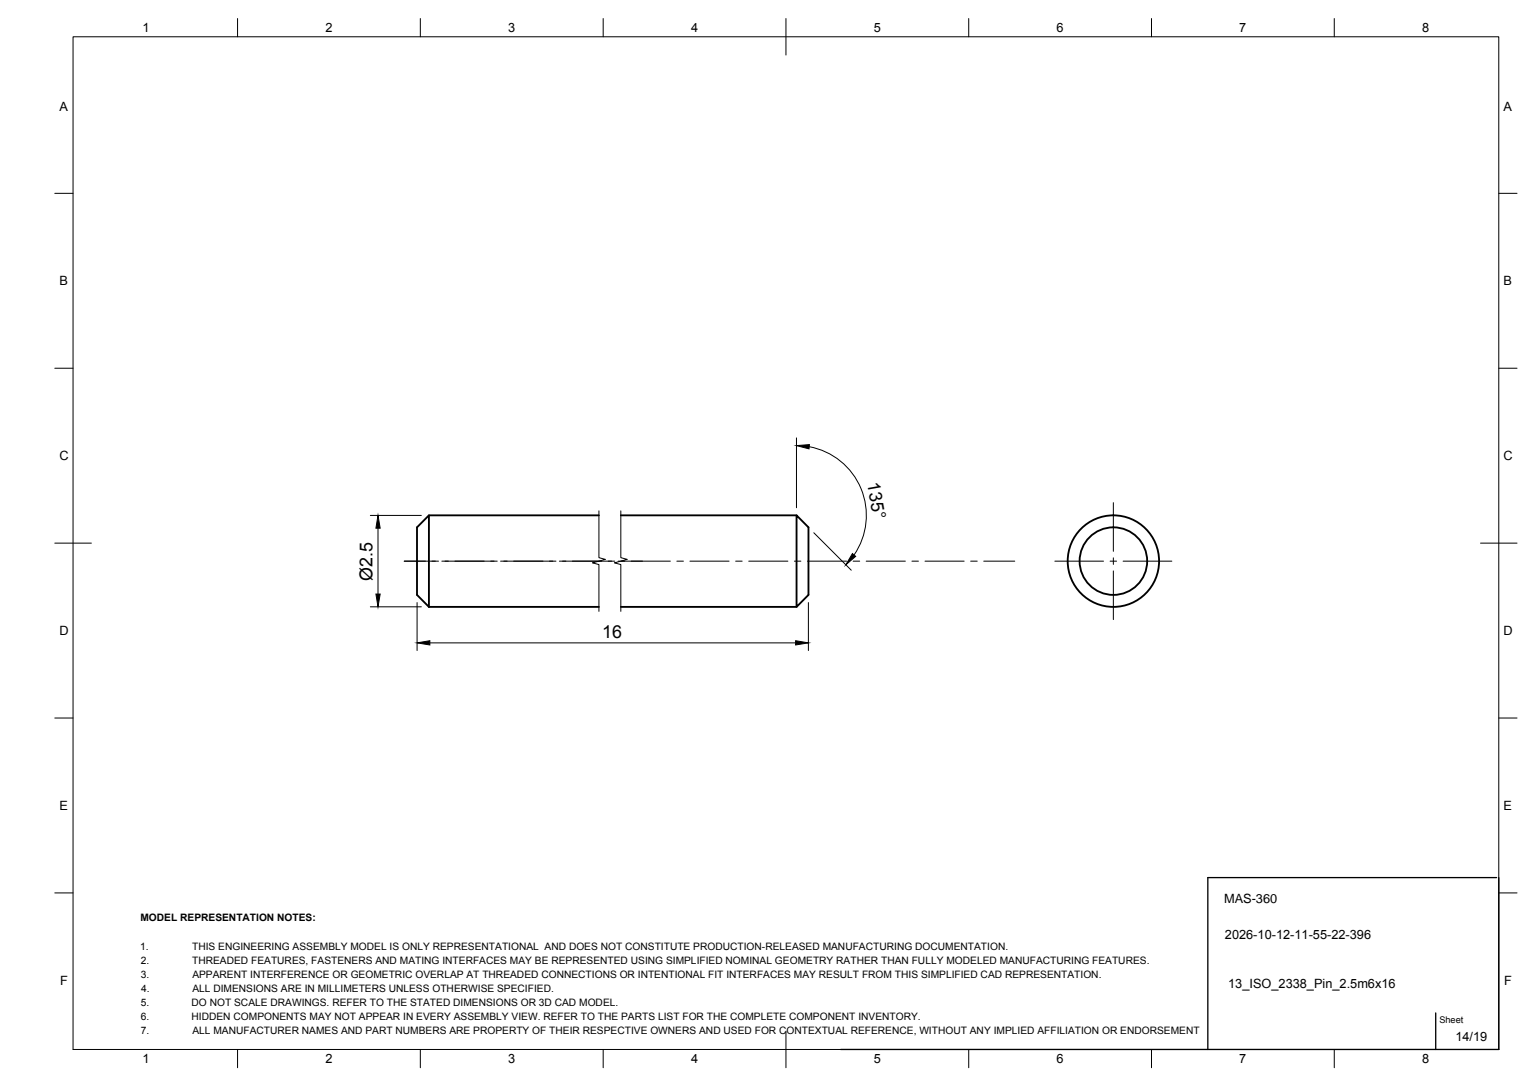
ISO-10303-21;
HEADER;
/* Generated by software containing ST-Developer
 * from STEP Tools, Inc. (www.steptools.com) 
 */

FILE_DESCRIPTION(
/* description */ (''),
/* implementation_level */ '2;1');

FILE_NAME(
/* name */ '13_ISO_2338_Pin_2.5m6x16.step',
/* time_stamp */ '2026-11-04T18:53:29-08:00',
/* author */ (''),
/* organization */ (''),
/* preprocessor_version */ 'ST-DEVELOPER v20.2',
/* originating_system */ 'Autodesk Translation Framework v15.17.0.0',
/* authorisation */ '');

FILE_SCHEMA (('AUTOMOTIVE_DESIGN { 1 0 10303 214 3 1 1 }'));
ENDSEC;

DATA;
#10=MECHANICAL_DESIGN_GEOMETRIC_PRESENTATION_REPRESENTATION('',(#1340),#100031);
#241=CONICAL_SURFACE('',#22428,1.0868,0.785398163397447);
#242=CONICAL_SURFACE('',#22433,1.0868,0.785398163397447);
#1152=CIRCLE('',#22429,1.25);
#1153=CIRCLE('',#22430,0.9236);
#1154=CIRCLE('',#22432,1.25);
#1155=CIRCLE('',#22434,0.9236);
#1304=SHAPE_REPRESENTATION_RELATIONSHIP('SRR','None',#100114,#1322);
#1322=ADVANCED_BREP_SHAPE_REPRESENTATION('',(#1358),#100026);
#1340=STYLED_ITEM('',(#100203),#1358);
#1358=MANIFOLD_SOLID_BREP('Body1',#20130);
#1679=PLANE('',#22435);
#1680=PLANE('',#22436);
#3248=LINE('',#99849,#4535);
#3249=LINE('',#99854,#4536);
#3250=LINE('',#99857,#4537);
#4535=VECTOR('',#27985,1.0868);
#4536=VECTOR('',#27992,1.25);
#4537=VECTOR('',#27995,1.0868);
#5016=CYLINDRICAL_SURFACE('',#22431,1.25);
#6147=FACE_OUTER_BOUND('',#7414,.T.);
#6148=FACE_OUTER_BOUND('',#7415,.T.);
#6149=FACE_OUTER_BOUND('',#7416,.T.);
#6150=FACE_OUTER_BOUND('',#7417,.T.);
#6151=FACE_OUTER_BOUND('',#7418,.T.);
#7414=EDGE_LOOP('',(#18749,#18750,#18751,#18752));
#7415=EDGE_LOOP('',(#18753,#18754,#18755,#18756));
#7416=EDGE_LOOP('',(#18757,#18758,#18759,#18760));
#7417=EDGE_LOOP('',(#18761));
#7418=EDGE_LOOP('',(#18762));
#9893=VERTEX_POINT('',#99846);
#9894=VERTEX_POINT('',#99848);
#9895=VERTEX_POINT('',#99852);
#9896=VERTEX_POINT('',#99856);
#12849=EDGE_CURVE('',#9893,#9893,#1152,.T.);
#12850=EDGE_CURVE('',#9893,#9894,#3248,.T.);
#12851=EDGE_CURVE('',#9894,#9894,#1153,.T.);
#12852=EDGE_CURVE('',#9895,#9895,#1154,.T.);
#12853=EDGE_CURVE('',#9895,#9893,#3249,.T.);
#12854=EDGE_CURVE('',#9895,#9896,#3250,.T.);
#12855=EDGE_CURVE('',#9896,#9896,#1155,.T.);
#18749=ORIENTED_EDGE('',*,*,#12849,.F.);
#18750=ORIENTED_EDGE('',*,*,#12850,.T.);
#18751=ORIENTED_EDGE('',*,*,#12851,.T.);
#18752=ORIENTED_EDGE('',*,*,#12850,.F.);
#18753=ORIENTED_EDGE('',*,*,#12852,.F.);
#18754=ORIENTED_EDGE('',*,*,#12853,.T.);
#18755=ORIENTED_EDGE('',*,*,#12849,.T.);
#18756=ORIENTED_EDGE('',*,*,#12853,.F.);
#18757=ORIENTED_EDGE('',*,*,#12852,.T.);
#18758=ORIENTED_EDGE('',*,*,#12854,.T.);
#18759=ORIENTED_EDGE('',*,*,#12855,.F.);
#18760=ORIENTED_EDGE('',*,*,#12854,.F.);
#18761=ORIENTED_EDGE('',*,*,#12855,.T.);
#18762=ORIENTED_EDGE('',*,*,#12851,.F.);
#20081=ADVANCED_FACE('',(#6147),#241,.T.);
#20082=ADVANCED_FACE('',(#6148),#5016,.T.);
#20083=ADVANCED_FACE('',(#6149),#242,.T.);
#20084=ADVANCED_FACE('',(#6150),#1679,.T.);
#20085=ADVANCED_FACE('',(#6151),#1680,.T.);
#20130=CLOSED_SHELL('',(#20081,#20082,#20083,#20084,#20085));
#22427=AXIS2_PLACEMENT_3D('',#99844,#27979,#27980);
#22428=AXIS2_PLACEMENT_3D('',#99845,#27981,#27982);
#22429=AXIS2_PLACEMENT_3D('',#99847,#27983,#27984);
#22430=AXIS2_PLACEMENT_3D('',#99850,#27986,#27987);
#22431=AXIS2_PLACEMENT_3D('',#99851,#27988,#27989);
#22432=AXIS2_PLACEMENT_3D('',#99853,#27990,#27991);
#22433=AXIS2_PLACEMENT_3D('',#99855,#27993,#27994);
#22434=AXIS2_PLACEMENT_3D('',#99858,#27996,#27997);
#22435=AXIS2_PLACEMENT_3D('',#99859,#27998,#27999);
#22436=AXIS2_PLACEMENT_3D('',#99860,#28000,#28001);
#27979=DIRECTION('axis',(0.,0.,1.));
#27980=DIRECTION('refdir',(1.,0.,0.));
#27981=DIRECTION('center_axis',(1.,0.,0.));
#27982=DIRECTION('ref_axis',(0.,1.,0.));
#27983=DIRECTION('center_axis',(1.,0.,0.));
#27984=DIRECTION('ref_axis',(0.,0.,-1.));
#27985=DIRECTION('',(-0.707106781186548,0.707106781186547,8.65956056235492E-17));
#27986=DIRECTION('center_axis',(1.,0.,0.));
#27987=DIRECTION('ref_axis',(0.,0.,-1.));
#27988=DIRECTION('center_axis',(1.,0.,0.));
#27989=DIRECTION('ref_axis',(0.,1.,0.));
#27990=DIRECTION('center_axis',(1.,0.,0.));
#27991=DIRECTION('ref_axis',(0.,0.,-1.));
#27992=DIRECTION('',(-1.,0.,0.));
#27993=DIRECTION('center_axis',(-1.,0.,0.));
#27994=DIRECTION('ref_axis',(0.,1.,0.));
#27995=DIRECTION('',(0.707106781186548,0.707106781186547,-8.65956056235492E-17));
#27996=DIRECTION('center_axis',(1.,0.,0.));
#27997=DIRECTION('ref_axis',(0.,0.,-1.));
#27998=DIRECTION('center_axis',(1.,0.,0.));
#27999=DIRECTION('ref_axis',(0.,0.,-1.));
#28000=DIRECTION('center_axis',(-1.,0.,0.));
#28001=DIRECTION('ref_axis',(0.,0.,1.));
#99844=CARTESIAN_POINT('',(0.,0.,0.));
#99845=CARTESIAN_POINT('Origin',(-7.8368,0.,0.));
#99846=CARTESIAN_POINT('',(-7.6736,-1.25,-1.53080849893419E-16));
#99847=CARTESIAN_POINT('Origin',(-7.6736,0.,0.));
#99848=CARTESIAN_POINT('',(-8.,-0.9236,-1.1310837836925E-16));
#99849=CARTESIAN_POINT('',(-7.8368,-1.0868,-1.33094614131334E-16));
#99850=CARTESIAN_POINT('Origin',(-8.,0.,0.));
#99851=CARTESIAN_POINT('Origin',(0.,0.,0.));
#99852=CARTESIAN_POINT('',(7.6736,-1.25,-1.53080849893419E-16));
#99853=CARTESIAN_POINT('Origin',(7.6736,0.,0.));
#99854=CARTESIAN_POINT('',(0.,-1.25,-1.53080849893419E-16));
#99855=CARTESIAN_POINT('Origin',(7.8368,0.,0.));
#99856=CARTESIAN_POINT('',(8.,-0.9236,-1.1310837836925E-16));
#99857=CARTESIAN_POINT('',(7.8368,-1.0868,1.33094614131334E-16));
#99858=CARTESIAN_POINT('Origin',(8.,0.,0.));
#99859=CARTESIAN_POINT('Origin',(8.,0.,0.));
#99860=CARTESIAN_POINT('Origin',(-8.,0.9236,0.));
#100006=UNCERTAINTY_MEASURE_WITH_UNIT(LENGTH_MEASURE(0.01),#100032,
'DISTANCE_ACCURACY_VALUE',
'Maximum model space distance between geometric entities at asserted c
onnectivities');
#100011=UNCERTAINTY_MEASURE_WITH_UNIT(LENGTH_MEASURE(0.01),#100032,
'DISTANCE_ACCURACY_VALUE',
'Maximum model space distance between geometric entities at asserted c
onnectivities');
#100026=(
GEOMETRIC_REPRESENTATION_CONTEXT(3)
GLOBAL_UNCERTAINTY_ASSIGNED_CONTEXT((#100006))
GLOBAL_UNIT_ASSIGNED_CONTEXT((#100032,#100034,#100035))
REPRESENTATION_CONTEXT('','3D')
);
#100031=(
GEOMETRIC_REPRESENTATION_CONTEXT(3)
GLOBAL_UNCERTAINTY_ASSIGNED_CONTEXT((#100011))
GLOBAL_UNIT_ASSIGNED_CONTEXT((#100032,#100034,#100035))
REPRESENTATION_CONTEXT('','3D')
);
#100032=(
LENGTH_UNIT()
NAMED_UNIT(*)
SI_UNIT(.MILLI.,.METRE.)
);
#100034=(
NAMED_UNIT(*)
PLANE_ANGLE_UNIT()
SI_UNIT($,.RADIAN.)
);
#100035=(
NAMED_UNIT(*)
SI_UNIT($,.STERADIAN.)
SOLID_ANGLE_UNIT()
);
#100050=SHAPE_DEFINITION_REPRESENTATION(#100069,#100114);
#100069=PRODUCT_DEFINITION_SHAPE('',$,#100134);
#100114=SHAPE_REPRESENTATION('',(#22427),#100026);
#100119=PRODUCT_DEFINITION_CONTEXT('part definition',#100178,'design');
#100134=PRODUCT_DEFINITION('2026-10-12-11-55-22-396',
'13_ISO_2338_Pin_2.5m6x16',#100153,#100119);
#100153=PRODUCT_DEFINITION_FORMATION('',$,#100194);
#100178=APPLICATION_CONTEXT(
'Core Data for Automotive Mechanical Design Process');
#100179=PRODUCT_CONTEXT('part definition',#100178,'mechanical');
#100194=PRODUCT('2026-10-12-11-55-22-396','13_ISO_2338_Pin_2.5m6x16',$,
(#100179));
#100203=PRESENTATION_STYLE_ASSIGNMENT((#100209));
#100209=SURFACE_STYLE_USAGE(.BOTH.,#100215);
#100215=SURFACE_SIDE_STYLE('',(#100221));
#100221=SURFACE_STYLE_FILL_AREA(#100227);
#100227=FILL_AREA_STYLE('Opaque(122,133,145)',(#100233));
#100233=FILL_AREA_STYLE_COLOUR('Opaque(122,133,145)',#100239);
#100239=COLOUR_RGB('Opaque(122,133,145)',0.47843137254902,0.52156862745098,
0.568627450980392);
ENDSEC;
END-ISO-10303-21;
